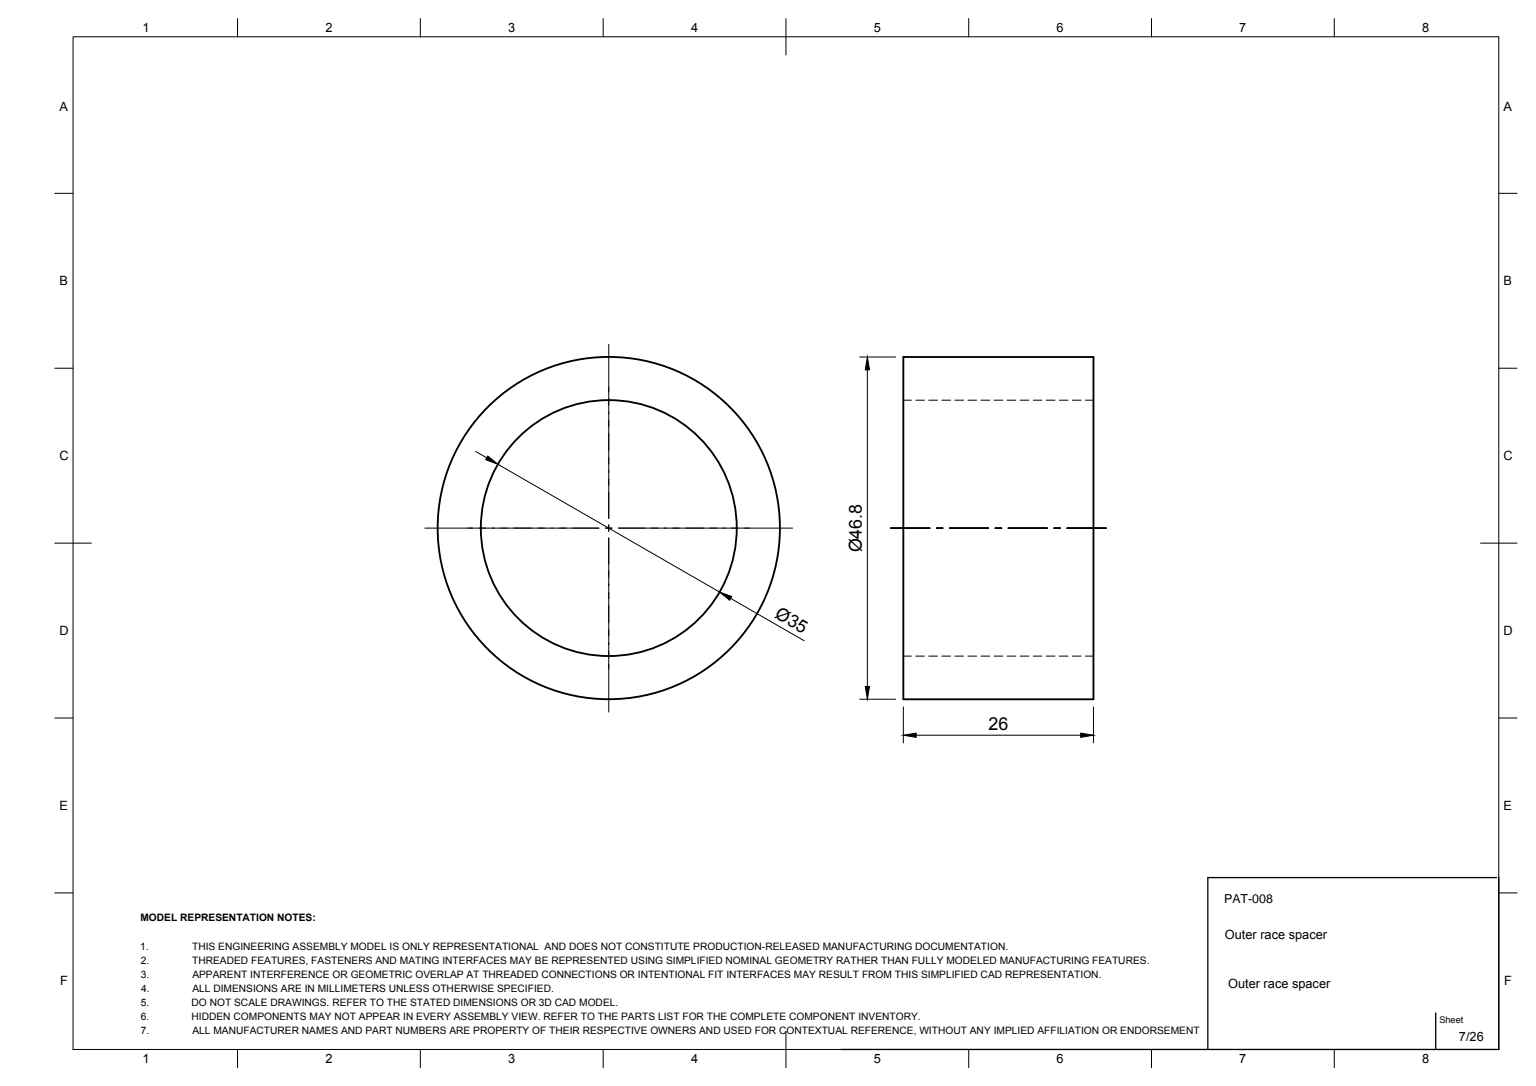
ISO-10303-21;
HEADER;
/* Generated by software containing ST-Developer
 * from STEP Tools, Inc. (www.steptools.com) 
 */

FILE_DESCRIPTION(
/* description */ ('Bearing housing with oil seal and end cap'),
/* implementation_level */ '2;1');

FILE_NAME(
/* name */ 'Outer race spacer.step',
/* time_stamp */ '2026-10-28T03:23:10-07:00',
/* author */ (''),
/* organization */ (''),
/* preprocessor_version */ 'ST-DEVELOPER v20.2',
/* originating_system */ 'Autodesk Translation Framework v15.17.0.0',
/* authorisation */ '');

FILE_SCHEMA (('AUTOMOTIVE_DESIGN { 1 0 10303 214 3 1 1 }'));
ENDSEC;

DATA;
#10=MECHANICAL_DESIGN_GEOMETRIC_PRESENTATION_REPRESENTATION('',(#261),#7871);
#219=SHAPE_REPRESENTATION_RELATIONSHIP('SRR','None',#7966,#240);
#240=ADVANCED_BREP_SHAPE_REPRESENTATION('',(#290),#7850);
#261=STYLED_ITEM('',(#8153),#290);
#290=MANIFOLD_SOLID_BREP('Body1',#4087);
#343=FACE_BOUND('',#886,.T.);
#344=FACE_BOUND('',#888,.T.);
#442=PLANE('',#4455);
#443=PLANE('',#4456);
#604=FACE_OUTER_BOUND('',#883,.T.);
#605=FACE_OUTER_BOUND('',#884,.T.);
#606=FACE_OUTER_BOUND('',#885,.T.);
#607=FACE_OUTER_BOUND('',#887,.T.);
#883=EDGE_LOOP('',(#2963,#2964,#2965,#2966));
#884=EDGE_LOOP('',(#2967,#2968,#2969,#2970));
#885=EDGE_LOOP('',(#2971));
#886=EDGE_LOOP('',(#2972));
#887=EDGE_LOOP('',(#2973));
#888=EDGE_LOOP('',(#2974));
#1213=LINE('',#6449,#1475);
#1214=LINE('',#6455,#1476);
#1475=VECTOR('',#5152,1.75);
#1476=VECTOR('',#5159,2.34);
#1715=CIRCLE('',#4450,1.75);
#1716=CIRCLE('',#4451,1.75);
#1717=CIRCLE('',#4453,2.34);
#1718=CIRCLE('',#4454,2.34);
#1963=VERTEX_POINT('',#6446);
#1964=VERTEX_POINT('',#6448);
#1965=VERTEX_POINT('',#6452);
#1966=VERTEX_POINT('',#6454);
#2345=EDGE_CURVE('',#1963,#1963,#1715,.T.);
#2346=EDGE_CURVE('',#1963,#1964,#1213,.T.);
#2347=EDGE_CURVE('',#1964,#1964,#1716,.T.);
#2348=EDGE_CURVE('',#1965,#1965,#1717,.T.);
#2349=EDGE_CURVE('',#1965,#1966,#1214,.T.);
#2350=EDGE_CURVE('',#1966,#1966,#1718,.T.);
#2963=ORIENTED_EDGE('',*,*,#2345,.F.);
#2964=ORIENTED_EDGE('',*,*,#2346,.T.);
#2965=ORIENTED_EDGE('',*,*,#2347,.T.);
#2966=ORIENTED_EDGE('',*,*,#2346,.F.);
#2967=ORIENTED_EDGE('',*,*,#2348,.F.);
#2968=ORIENTED_EDGE('',*,*,#2349,.T.);
#2969=ORIENTED_EDGE('',*,*,#2350,.T.);
#2970=ORIENTED_EDGE('',*,*,#2349,.F.);
#2971=ORIENTED_EDGE('',*,*,#2348,.T.);
#2972=ORIENTED_EDGE('',*,*,#2345,.T.);
#2973=ORIENTED_EDGE('',*,*,#2350,.F.);
#2974=ORIENTED_EDGE('',*,*,#2347,.F.);
#3777=CYLINDRICAL_SURFACE('',#4449,1.75);
#3778=CYLINDRICAL_SURFACE('',#4452,2.34);
#3886=ADVANCED_FACE('',(#604),#3777,.F.);
#3887=ADVANCED_FACE('',(#605),#3778,.T.);
#3888=ADVANCED_FACE('',(#606,#343),#442,.T.);
#3889=ADVANCED_FACE('',(#607,#344),#443,.F.);
#4087=CLOSED_SHELL('',(#3886,#3887,#3888,#3889));
#4448=AXIS2_PLACEMENT_3D('',#6444,#5146,#5147);
#4449=AXIS2_PLACEMENT_3D('',#6445,#5148,#5149);
#4450=AXIS2_PLACEMENT_3D('',#6447,#5150,#5151);
#4451=AXIS2_PLACEMENT_3D('',#6450,#5153,#5154);
#4452=AXIS2_PLACEMENT_3D('',#6451,#5155,#5156);
#4453=AXIS2_PLACEMENT_3D('',#6453,#5157,#5158);
#4454=AXIS2_PLACEMENT_3D('',#6456,#5160,#5161);
#4455=AXIS2_PLACEMENT_3D('',#6457,#5162,#5163);
#4456=AXIS2_PLACEMENT_3D('',#6458,#5164,#5165);
#5146=DIRECTION('axis',(0.,0.,1.));
#5147=DIRECTION('refdir',(1.,0.,0.));
#5148=DIRECTION('center_axis',(0.,1.,0.));
#5149=DIRECTION('ref_axis',(1.,0.,0.));
#5150=DIRECTION('center_axis',(0.,-1.,0.));
#5151=DIRECTION('ref_axis',(1.,0.,0.));
#5152=DIRECTION('',(0.,-1.,0.));
#5153=DIRECTION('center_axis',(0.,-1.,0.));
#5154=DIRECTION('ref_axis',(1.,0.,0.));
#5155=DIRECTION('center_axis',(0.,1.,0.));
#5156=DIRECTION('ref_axis',(1.,0.,0.));
#5157=DIRECTION('center_axis',(0.,1.,0.));
#5158=DIRECTION('ref_axis',(1.,0.,0.));
#5159=DIRECTION('',(0.,-1.,0.));
#5160=DIRECTION('center_axis',(0.,1.,0.));
#5161=DIRECTION('ref_axis',(1.,0.,0.));
#5162=DIRECTION('center_axis',(0.,1.,0.));
#5163=DIRECTION('ref_axis',(1.,0.,0.));
#5164=DIRECTION('center_axis',(0.,1.,0.));
#5165=DIRECTION('ref_axis',(1.,0.,0.));
#6444=CARTESIAN_POINT('',(0.,0.,0.));
#6445=CARTESIAN_POINT('Origin',(0.,1.7,4.5));
#6446=CARTESIAN_POINT('',(-1.75,4.3,4.5));
#6447=CARTESIAN_POINT('Origin',(0.,4.3,4.5));
#6448=CARTESIAN_POINT('',(-1.75,1.7,4.5));
#6449=CARTESIAN_POINT('',(-1.75,1.7,4.5));
#6450=CARTESIAN_POINT('Origin',(0.,1.7,4.5));
#6451=CARTESIAN_POINT('Origin',(0.,1.7,4.5));
#6452=CARTESIAN_POINT('',(-2.34,4.3,4.5));
#6453=CARTESIAN_POINT('Origin',(0.,4.3,4.5));
#6454=CARTESIAN_POINT('',(-2.34,1.7,4.5));
#6455=CARTESIAN_POINT('',(-2.34,1.7,4.5));
#6456=CARTESIAN_POINT('Origin',(0.,1.7,4.5));
#6457=CARTESIAN_POINT('Origin',(0.,4.3,4.5));
#6458=CARTESIAN_POINT('Origin',(0.,1.7,4.5));
#7824=UNCERTAINTY_MEASURE_WITH_UNIT(LENGTH_MEASURE(0.001),#7872,
'DISTANCE_ACCURACY_VALUE',
'Maximum model space distance between geometric entities at asserted c
onnectivities');
#7845=UNCERTAINTY_MEASURE_WITH_UNIT(LENGTH_MEASURE(0.001),#7872,
'DISTANCE_ACCURACY_VALUE',
'Maximum model space distance between geometric entities at asserted c
onnectivities');
#7850=(
GEOMETRIC_REPRESENTATION_CONTEXT(3)
GLOBAL_UNCERTAINTY_ASSIGNED_CONTEXT((#7824))
GLOBAL_UNIT_ASSIGNED_CONTEXT((#7872,#7874,#7875))
REPRESENTATION_CONTEXT('','3D')
);
#7871=(
GEOMETRIC_REPRESENTATION_CONTEXT(3)
GLOBAL_UNCERTAINTY_ASSIGNED_CONTEXT((#7845))
GLOBAL_UNIT_ASSIGNED_CONTEXT((#7872,#7874,#7875))
REPRESENTATION_CONTEXT('','3D')
);
#7872=(
LENGTH_UNIT()
NAMED_UNIT(*)
SI_UNIT(.CENTI.,.METRE.)
);
#7874=(
NAMED_UNIT(*)
PLANE_ANGLE_UNIT()
SI_UNIT($,.RADIAN.)
);
#7875=(
NAMED_UNIT(*)
SI_UNIT($,.STERADIAN.)
SOLID_ANGLE_UNIT()
);
#7880=SHAPE_DEFINITION_REPRESENTATION(#7905,#7966);
#7905=PRODUCT_DEFINITION_SHAPE('',$,#7992);
#7966=SHAPE_REPRESENTATION('',(#4448),#7850);
#7987=PRODUCT_DEFINITION_CONTEXT('part definition',#8064,'design');
#7992=PRODUCT_DEFINITION('Outer race spacer','Outer race spacer',#8017,
#7987);
#8017=PRODUCT_DEFINITION_FORMATION('',$,#8070);
#8064=APPLICATION_CONTEXT(
'Core Data for Automotive Mechanical Design Process');
#8065=PRODUCT_CONTEXT('part definition',#8064,'mechanical');
#8070=PRODUCT('Outer race spacer','Outer race spacer',
'Outer race spacer',(#8065));
#8147=COLOUR_RGB('Grey',0.48,0.52,0.57);
#8148=FILL_AREA_STYLE_COLOUR('',#8147);
#8149=FILL_AREA_STYLE('',(#8148));
#8150=SURFACE_STYLE_FILL_AREA(#8149);
#8151=SURFACE_SIDE_STYLE('',(#8150));
#8152=SURFACE_STYLE_USAGE(.BOTH.,#8151);
#8153=PRESENTATION_STYLE_ASSIGNMENT((#8152));
ENDSEC;
END-ISO-10303-21;
